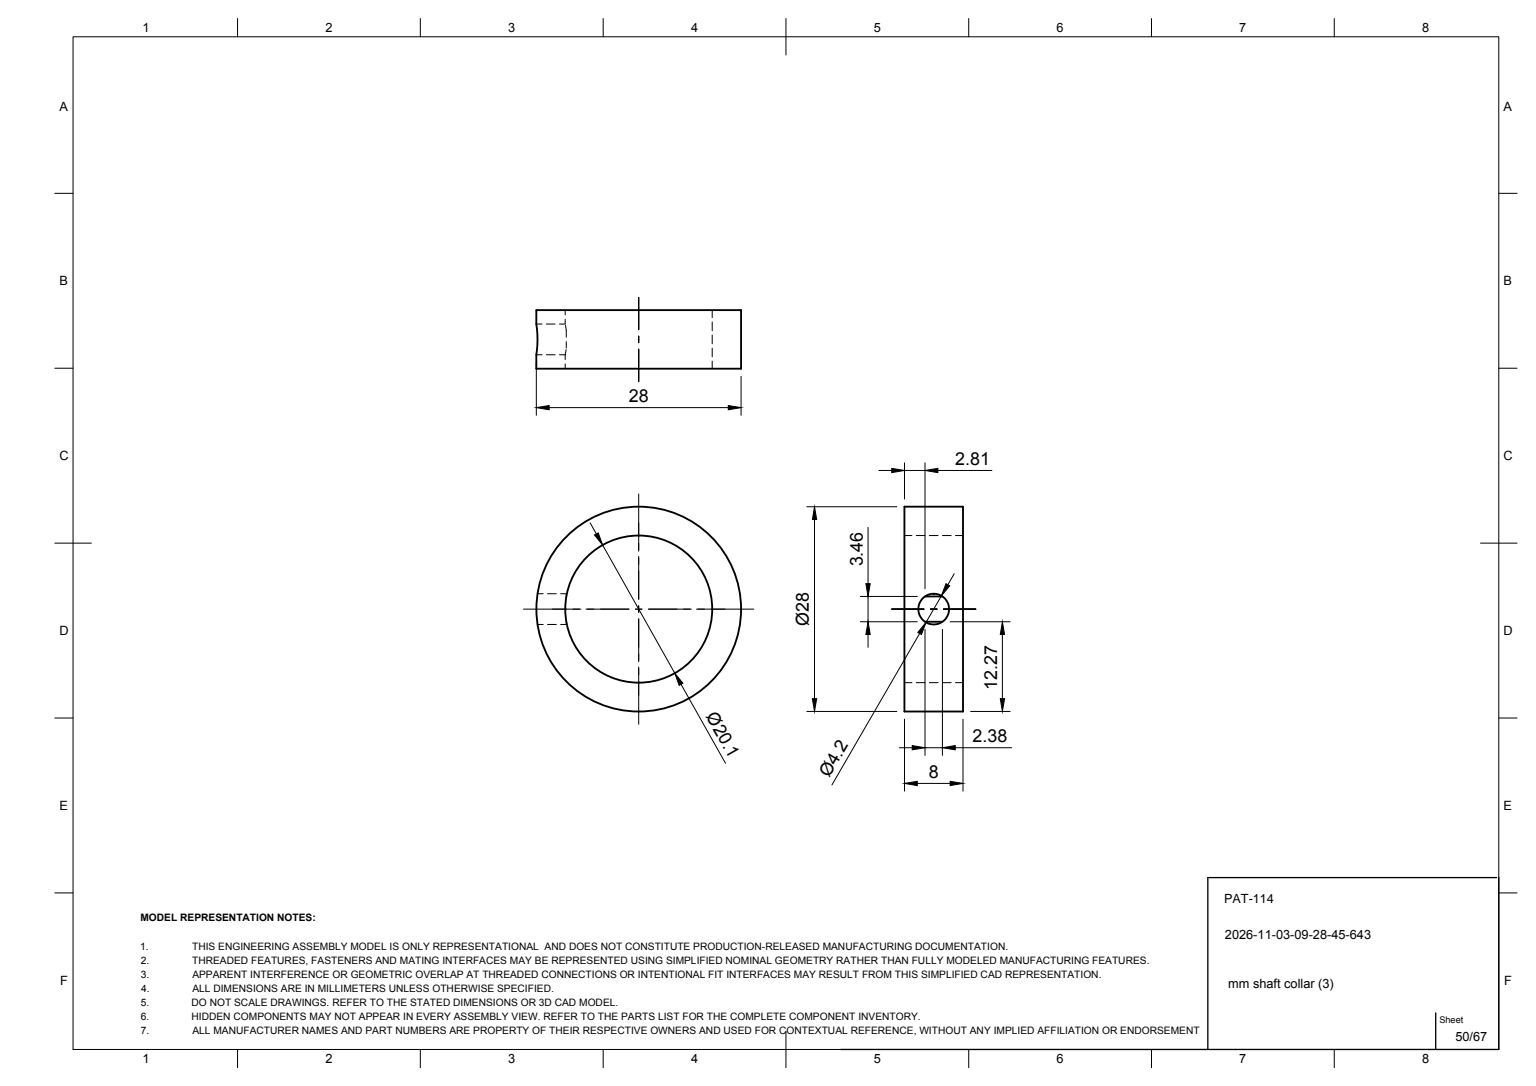
ISO-10303-21;
HEADER;
/* Generated by software containing ST-Developer
 * from STEP Tools, Inc. (www.steptools.com) 
 */

FILE_DESCRIPTION(
/* description */ ('Two-stage gear reducer in split housing'),
/* implementation_level */ '2;1');

FILE_NAME(
/* name */ 'mm shaft collar (3).step',
/* time_stamp */ '2026-10-28T03:22:31-07:00',
/* author */ (''),
/* organization */ (''),
/* preprocessor_version */ 'ST-DEVELOPER v20.2',
/* originating_system */ 'Autodesk Translation Framework v15.17.0.0',
/* authorisation */ '');

FILE_SCHEMA (('AUTOMOTIVE_DESIGN { 1 0 10303 214 3 1 1 }'));
ENDSEC;

DATA;
#10=MECHANICAL_DESIGN_GEOMETRIC_PRESENTATION_REPRESENTATION('',(#1288),#73366);
#975=B_SPLINE_CURVE_WITH_KNOTS('',3,(#37499,#37500,#37501,#37502,#37503,
#37504,#37505,#37506,#37507,#37508,#37509,#37510,#37511,#37512),
 .UNSPECIFIED.,.F.,.F.,(4,2,2,2,2,2,4),(0.75600573798703,0.793568827564647,
0.872922520054202,0.952276212543757,1.03162990503331,1.11098359752287,1.14854668710048),
 .UNSPECIFIED.);
#976=B_SPLINE_CURVE_WITH_KNOTS('',3,(#37518,#37519,#37520,#37521,#37522,
#37523,#37524,#37525,#37526,#37527,#37528,#37529,#37530,#37531,#37532,#37533,
#37534,#37535),.UNSPECIFIED.,.F.,.F.,(4,2,2,2,2,2,2,2,4),(0.,0.0792334805614374,
0.158466961122875,0.237699060165218,0.31693115920756,0.396163258249903,
0.475395357292246,0.554628837853684,0.633862318415121),.UNSPECIFIED.);
#977=B_SPLINE_CURVE_WITH_KNOTS('',3,(#37536,#37537,#37538,#37539,#37540,
#37541,#37542,#37543,#37544,#37545,#37546,#37547,#37548,#37549,#37550,#37551,
#37552,#37553),.UNSPECIFIED.,.F.,.F.,(4,2,2,2,2,2,2,2,4),(0.633862318415121,
0.713095798976559,0.792329279537996,0.871561378580339,0.950793477622681,
1.03002557666502,1.10925767570737,1.1884911562688,1.26772463683024),
 .UNSPECIFIED.);
#978=B_SPLINE_CURVE_WITH_KNOTS('',3,(#37556,#37557,#37558,#37559,#37560,
#37561,#37562,#37563,#37564,#37565,#37566,#37567,#37568,#37569),
 .UNSPECIFIED.,.F.,.F.,(4,2,2,2,2,2,4),(0.121154929624528,0.158718019202143,
0.238071711691698,0.317425404181252,0.396779096670807,0.476132789160361,
0.513695878737976),.UNSPECIFIED.);
#1161=SHAPE_REPRESENTATION_RELATIONSHIP('SRR','None',#73652,#1217);
#1217=ADVANCED_BREP_SHAPE_REPRESENTATION('',(#1357),#73348);
#1288=STYLED_ITEM('',(#73988),#1357);
#1357=MANIFOLD_SOLID_BREP('Body1',#16178);
#1564=FACE_BOUND('',#3679,.T.);
#1565=FACE_BOUND('',#3681,.T.);
#1566=FACE_BOUND('',#3683,.T.);
#1567=FACE_BOUND('',#3685,.T.);
#1874=PLANE('',#17985);
#1875=PLANE('',#17990);
#1876=PLANE('',#17997);
#1877=PLANE('',#17998);
#2572=FACE_OUTER_BOUND('',#3675,.T.);
#2573=FACE_OUTER_BOUND('',#3676,.T.);
#2574=FACE_OUTER_BOUND('',#3677,.T.);
#2575=FACE_OUTER_BOUND('',#3678,.T.);
#2576=FACE_OUTER_BOUND('',#3680,.T.);
#2577=FACE_OUTER_BOUND('',#3682,.T.);
#2578=FACE_OUTER_BOUND('',#3684,.T.);
#3675=EDGE_LOOP('',(#13075,#13076));
#3676=EDGE_LOOP('',(#13077,#13078,#13079,#13080,#13081,#13082,#13083,#13084,
#13085));
#3677=EDGE_LOOP('',(#13086,#13087,#13088));
#3678=EDGE_LOOP('',(#13089,#13090,#13091,#13092));
#3679=EDGE_LOOP('',(#13093,#13094,#13095,#13096));
#3680=EDGE_LOOP('',(#13097,#13098,#13099,#13100));
#3681=EDGE_LOOP('',(#13101,#13102));
#3682=EDGE_LOOP('',(#13103));
#3683=EDGE_LOOP('',(#13104));
#3684=EDGE_LOOP('',(#13105));
#3685=EDGE_LOOP('',(#13106));
#4689=LINE('',#37495,#5713);
#4690=LINE('',#37516,#5714);
#4691=LINE('',#37571,#5715);
#4692=LINE('',#37576,#5716);
#4693=LINE('',#37582,#5717);
#5713=VECTOR('',#21439,1.);
#5714=VECTOR('',#21446,0.21);
#5715=VECTOR('',#21451,1.);
#5716=VECTOR('',#21456,1.005);
#5717=VECTOR('',#21463,1.4);
#6631=CIRCLE('',#17986,0.21);
#6632=CIRCLE('',#17988,0.21);
#6633=CIRCLE('',#17989,0.21);
#6634=CIRCLE('',#17992,1.005);
#6635=CIRCLE('',#17993,1.005);
#6636=CIRCLE('',#17995,1.4);
#6637=CIRCLE('',#17996,1.4);
#7696=VERTEX_POINT('',#37493);
#7697=VERTEX_POINT('',#37494);
#7698=VERTEX_POINT('',#37498);
#7699=VERTEX_POINT('',#37513);
#7700=VERTEX_POINT('',#37515);
#7701=VERTEX_POINT('',#37517);
#7702=VERTEX_POINT('',#37554);
#7703=VERTEX_POINT('',#37573);
#7704=VERTEX_POINT('',#37575);
#7705=VERTEX_POINT('',#37579);
#7706=VERTEX_POINT('',#37581);
#9591=EDGE_CURVE('',#7696,#7697,#4689,.T.);
#9592=EDGE_CURVE('',#7696,#7697,#6631,.T.);
#9593=EDGE_CURVE('',#7698,#7696,#975,.T.);
#9594=EDGE_CURVE('',#7699,#7698,#6632,.T.);
#9595=EDGE_CURVE('',#7699,#7700,#4690,.T.);
#9596=EDGE_CURVE('',#7701,#7700,#976,.T.);
#9597=EDGE_CURVE('',#7700,#7701,#977,.T.);
#9598=EDGE_CURVE('',#7702,#7699,#6633,.T.);
#9599=EDGE_CURVE('',#7697,#7702,#978,.T.);
#9600=EDGE_CURVE('',#7702,#7698,#4691,.T.);
#9601=EDGE_CURVE('',#7703,#7703,#6634,.T.);
#9602=EDGE_CURVE('',#7703,#7704,#4692,.T.);
#9603=EDGE_CURVE('',#7704,#7704,#6635,.T.);
#9604=EDGE_CURVE('',#7705,#7705,#6636,.T.);
#9605=EDGE_CURVE('',#7705,#7706,#4693,.T.);
#9606=EDGE_CURVE('',#7706,#7706,#6637,.T.);
#13075=ORIENTED_EDGE('',*,*,#9591,.F.);
#13076=ORIENTED_EDGE('',*,*,#9592,.T.);
#13077=ORIENTED_EDGE('',*,*,#9593,.F.);
#13078=ORIENTED_EDGE('',*,*,#9594,.F.);
#13079=ORIENTED_EDGE('',*,*,#9595,.T.);
#13080=ORIENTED_EDGE('',*,*,#9596,.F.);
#13081=ORIENTED_EDGE('',*,*,#9597,.F.);
#13082=ORIENTED_EDGE('',*,*,#9595,.F.);
#13083=ORIENTED_EDGE('',*,*,#9598,.F.);
#13084=ORIENTED_EDGE('',*,*,#9599,.F.);
#13085=ORIENTED_EDGE('',*,*,#9592,.F.);
#13086=ORIENTED_EDGE('',*,*,#9600,.F.);
#13087=ORIENTED_EDGE('',*,*,#9598,.T.);
#13088=ORIENTED_EDGE('',*,*,#9594,.T.);
#13089=ORIENTED_EDGE('',*,*,#9601,.F.);
#13090=ORIENTED_EDGE('',*,*,#9602,.T.);
#13091=ORIENTED_EDGE('',*,*,#9603,.T.);
#13092=ORIENTED_EDGE('',*,*,#9602,.F.);
#13093=ORIENTED_EDGE('',*,*,#9599,.T.);
#13094=ORIENTED_EDGE('',*,*,#9600,.T.);
#13095=ORIENTED_EDGE('',*,*,#9593,.T.);
#13096=ORIENTED_EDGE('',*,*,#9591,.T.);
#13097=ORIENTED_EDGE('',*,*,#9604,.F.);
#13098=ORIENTED_EDGE('',*,*,#9605,.T.);
#13099=ORIENTED_EDGE('',*,*,#9606,.T.);
#13100=ORIENTED_EDGE('',*,*,#9605,.F.);
#13101=ORIENTED_EDGE('',*,*,#9596,.T.);
#13102=ORIENTED_EDGE('',*,*,#9597,.T.);
#13103=ORIENTED_EDGE('',*,*,#9604,.T.);
#13104=ORIENTED_EDGE('',*,*,#9601,.T.);
#13105=ORIENTED_EDGE('',*,*,#9606,.F.);
#13106=ORIENTED_EDGE('',*,*,#9603,.F.);
#15116=CYLINDRICAL_SURFACE('',#17987,0.21);
#15117=CYLINDRICAL_SURFACE('',#17991,1.005);
#15118=CYLINDRICAL_SURFACE('',#17994,1.4);
#15779=ADVANCED_FACE('',(#2572),#1874,.T.);
#15780=ADVANCED_FACE('',(#2573),#15116,.F.);
#15781=ADVANCED_FACE('',(#2574),#1875,.T.);
#15782=ADVANCED_FACE('',(#2575,#1564),#15117,.F.);
#15783=ADVANCED_FACE('',(#2576,#1565),#15118,.T.);
#15784=ADVANCED_FACE('',(#2577,#1566),#1876,.T.);
#15785=ADVANCED_FACE('',(#2578,#1567),#1877,.F.);
#16178=CLOSED_SHELL('',(#15779,#15780,#15781,#15782,#15783,#15784,#15785));
#17984=AXIS2_PLACEMENT_3D('',#37491,#21435,#21436);
#17985=AXIS2_PLACEMENT_3D('',#37492,#21437,#21438);
#17986=AXIS2_PLACEMENT_3D('',#37496,#21440,#21441);
#17987=AXIS2_PLACEMENT_3D('',#37497,#21442,#21443);
#17988=AXIS2_PLACEMENT_3D('',#37514,#21444,#21445);
#17989=AXIS2_PLACEMENT_3D('',#37555,#21447,#21448);
#17990=AXIS2_PLACEMENT_3D('',#37570,#21449,#21450);
#17991=AXIS2_PLACEMENT_3D('',#37572,#21452,#21453);
#17992=AXIS2_PLACEMENT_3D('',#37574,#21454,#21455);
#17993=AXIS2_PLACEMENT_3D('',#37577,#21457,#21458);
#17994=AXIS2_PLACEMENT_3D('',#37578,#21459,#21460);
#17995=AXIS2_PLACEMENT_3D('',#37580,#21461,#21462);
#17996=AXIS2_PLACEMENT_3D('',#37583,#21464,#21465);
#17997=AXIS2_PLACEMENT_3D('',#37584,#21466,#21467);
#17998=AXIS2_PLACEMENT_3D('',#37585,#21468,#21469);
#21435=DIRECTION('axis',(0.,0.,1.));
#21436=DIRECTION('refdir',(1.,0.,0.));
#21437=DIRECTION('center_axis',(0.,0.,1.));
#21438=DIRECTION('ref_axis',(1.,0.,0.));
#21439=DIRECTION('',(0.,1.,0.));
#21440=DIRECTION('center_axis',(0.,0.,1.));
#21441=DIRECTION('ref_axis',(1.,0.,0.));
#21442=DIRECTION('center_axis',(0.,0.,1.));
#21443=DIRECTION('ref_axis',(1.,0.,0.));
#21444=DIRECTION('center_axis',(0.,0.,1.));
#21445=DIRECTION('ref_axis',(1.,0.,0.));
#21446=DIRECTION('',(0.,0.,1.));
#21447=DIRECTION('center_axis',(0.,0.,1.));
#21448=DIRECTION('ref_axis',(1.,0.,0.));
#21449=DIRECTION('center_axis',(0.,0.,1.));
#21450=DIRECTION('ref_axis',(1.,0.,0.));
#21451=DIRECTION('',(0.,-1.,0.));
#21452=DIRECTION('center_axis',(0.,1.,0.));
#21453=DIRECTION('ref_axis',(1.,0.,0.));
#21454=DIRECTION('center_axis',(0.,-1.,0.));
#21455=DIRECTION('ref_axis',(1.,0.,0.));
#21456=DIRECTION('',(0.,-1.,0.));
#21457=DIRECTION('center_axis',(0.,-1.,0.));
#21458=DIRECTION('ref_axis',(1.,0.,0.));
#21459=DIRECTION('center_axis',(0.,1.,0.));
#21460=DIRECTION('ref_axis',(1.,0.,0.));
#21461=DIRECTION('center_axis',(0.,1.,0.));
#21462=DIRECTION('ref_axis',(1.,0.,0.));
#21463=DIRECTION('',(0.,-1.,0.));
#21464=DIRECTION('center_axis',(0.,1.,0.));
#21465=DIRECTION('ref_axis',(1.,0.,0.));
#21466=DIRECTION('center_axis',(0.,1.,0.));
#21467=DIRECTION('ref_axis',(1.,0.,0.));
#21468=DIRECTION('center_axis',(0.,1.,0.));
#21469=DIRECTION('ref_axis',(1.,0.,0.));
#37491=CARTESIAN_POINT('',(0.,0.,0.));
#37492=CARTESIAN_POINT('Origin',(6.,8.2,10.99));
#37493=CARTESIAN_POINT('',(6.17298843892005,8.08094119100208,10.99));
#37494=CARTESIAN_POINT('',(6.17298843892005,8.31905880899792,10.99));
#37495=CARTESIAN_POINT('',(6.17298843892005,7.8,10.99));
#37496=CARTESIAN_POINT('Origin',(6.,8.2,10.99));
#37497=CARTESIAN_POINT('Origin',(6.,8.2,10.99));
#37498=CARTESIAN_POINT('',(5.82701156107995,8.08094119100208,10.99));
#37499=CARTESIAN_POINT('Ctrl Pts',(5.82701156107995,8.08094119100207,10.99));
#37500=CARTESIAN_POINT('Ctrl Pts',(5.83440513468869,8.0701985776047,10.9912919219764));
#37501=CARTESIAN_POINT('Ctrl Pts',(5.8427028612744,8.06031229062725,10.992653949439));
#37502=CARTESIAN_POINT('Ctrl Pts',(5.87010792615492,8.03290722574673,10.9967480843909));
#37503=CARTESIAN_POINT('Ctrl Pts',(5.89366983224071,8.01675794366705,10.9996958932764));
#37504=CARTESIAN_POINT('Ctrl Pts',(5.94538709536759,7.99530220603509,11.0038502947236));
#37505=CARTESIAN_POINT('Ctrl Pts',(5.97354876917015,7.99,11.005));
#37506=CARTESIAN_POINT('Ctrl Pts',(6.02645123082985,7.99,11.005));
#37507=CARTESIAN_POINT('Ctrl Pts',(6.05461290463241,7.99530220603509,11.0038502947236));
#37508=CARTESIAN_POINT('Ctrl Pts',(6.10633016775928,8.01675794366705,10.9996958932764));
#37509=CARTESIAN_POINT('Ctrl Pts',(6.12989207384508,8.03290722574673,10.9967480843909));
#37510=CARTESIAN_POINT('Ctrl Pts',(6.1572971387256,8.06031229062725,10.992653949439));
#37511=CARTESIAN_POINT('Ctrl Pts',(6.16559486531131,8.0701985776047,10.9912919219764));
#37512=CARTESIAN_POINT('Ctrl Pts',(6.17298843892005,8.08094119100208,10.99));
#37513=CARTESIAN_POINT('',(5.79,8.2,10.99));
#37514=CARTESIAN_POINT('Origin',(6.,8.2,10.99));
#37515=CARTESIAN_POINT('',(5.79,8.2,11.38416039533));
#37516=CARTESIAN_POINT('',(5.79,8.2,10.99));
#37517=CARTESIAN_POINT('',(6.21,8.2,11.38416039533));
#37518=CARTESIAN_POINT('Ctrl Pts',(6.21,8.2,11.38416039533));
#37519=CARTESIAN_POINT('Ctrl Pts',(6.21,8.17358883981285,11.38416039533));
#37520=CARTESIAN_POINT('Ctrl Pts',(6.20471354911189,8.1454449403829,11.3849944296993));
#37521=CARTESIAN_POINT('Ctrl Pts',(6.18326999585849,8.09371735000826,11.3879947099895));
#37522=CARTESIAN_POINT('Ctrl Pts',(6.16711503760643,8.07013018950807,11.3901162943626));
#37523=CARTESIAN_POINT('Ctrl Pts',(6.12987013519678,8.03288528709843,11.394089123191));
#37524=CARTESIAN_POINT('Ctrl Pts',(6.10628283459019,8.01673007414492,11.3962002442067));
#37525=CARTESIAN_POINT('Ctrl Pts',(6.05455476560391,7.99528633552708,11.3991765222353));
#37526=CARTESIAN_POINT('Ctrl Pts',(6.02641069968078,7.99,11.4));
#37527=CARTESIAN_POINT('Ctrl Pts',(5.97358930031922,7.99,11.4));
#37528=CARTESIAN_POINT('Ctrl Pts',(5.94544523439609,7.99528633552708,11.3991765222353));
#37529=CARTESIAN_POINT('Ctrl Pts',(5.89371716540981,8.01673007414492,11.3962002442067));
#37530=CARTESIAN_POINT('Ctrl Pts',(5.87012986480322,8.03288528709843,11.394089123191));
#37531=CARTESIAN_POINT('Ctrl Pts',(5.83288496239357,8.07013018950807,11.3901162943626));
#37532=CARTESIAN_POINT('Ctrl Pts',(5.81673000414151,8.09371735000826,11.3879947099895));
#37533=CARTESIAN_POINT('Ctrl Pts',(5.79528645088811,8.1454449403829,11.3849944296993));
#37534=CARTESIAN_POINT('Ctrl Pts',(5.79,8.17358883981285,11.38416039533));
#37535=CARTESIAN_POINT('Ctrl Pts',(5.79,8.2,11.38416039533));
#37536=CARTESIAN_POINT('Ctrl Pts',(5.79,8.2,11.38416039533));
#37537=CARTESIAN_POINT('Ctrl Pts',(5.79,8.22641116018715,11.38416039533));
#37538=CARTESIAN_POINT('Ctrl Pts',(5.79528645088811,8.2545550596171,11.3849944296993));
#37539=CARTESIAN_POINT('Ctrl Pts',(5.81673000414151,8.30628264999174,11.3879947099895));
#37540=CARTESIAN_POINT('Ctrl Pts',(5.83288496239357,8.32986981049192,11.3901162943626));
#37541=CARTESIAN_POINT('Ctrl Pts',(5.87012986480322,8.36711471290156,11.394089123191));
#37542=CARTESIAN_POINT('Ctrl Pts',(5.89371716540981,8.38326992585508,11.3962002442067));
#37543=CARTESIAN_POINT('Ctrl Pts',(5.94544523439609,8.40471366447292,11.3991765222353));
#37544=CARTESIAN_POINT('Ctrl Pts',(5.97358930031922,8.41,11.4));
#37545=CARTESIAN_POINT('Ctrl Pts',(6.02641069968078,8.41,11.4));
#37546=CARTESIAN_POINT('Ctrl Pts',(6.05455476560391,8.40471366447292,11.3991765222353));
#37547=CARTESIAN_POINT('Ctrl Pts',(6.10628283459019,8.38326992585508,11.3962002442067));
#37548=CARTESIAN_POINT('Ctrl Pts',(6.12987013519678,8.36711471290156,11.394089123191));
#37549=CARTESIAN_POINT('Ctrl Pts',(6.16711503760642,8.32986981049192,11.3901162943626));
#37550=CARTESIAN_POINT('Ctrl Pts',(6.18326999585849,8.30628264999174,11.3879947099895));
#37551=CARTESIAN_POINT('Ctrl Pts',(6.2047135491119,8.2545550596171,11.3849944296993));
#37552=CARTESIAN_POINT('Ctrl Pts',(6.21,8.22641116018714,11.38416039533));
#37553=CARTESIAN_POINT('Ctrl Pts',(6.21,8.2,11.38416039533));
#37554=CARTESIAN_POINT('',(5.82701156107995,8.31905880899792,10.99));
#37555=CARTESIAN_POINT('Origin',(6.,8.2,10.99));
#37556=CARTESIAN_POINT('Ctrl Pts',(6.17298843892005,8.31905880899792,10.99));
#37557=CARTESIAN_POINT('Ctrl Pts',(6.16559486531131,8.3298014223953,10.9912919219764));
#37558=CARTESIAN_POINT('Ctrl Pts',(6.1572971387256,8.33968770937275,10.992653949439));
#37559=CARTESIAN_POINT('Ctrl Pts',(6.12989207384508,8.36709277425327,10.9967480843909));
#37560=CARTESIAN_POINT('Ctrl Pts',(6.10633016775928,8.38324205633295,10.9996958932764));
#37561=CARTESIAN_POINT('Ctrl Pts',(6.05461290463241,8.40469779396491,11.0038502947236));
#37562=CARTESIAN_POINT('Ctrl Pts',(6.02645123082985,8.41,11.005));
#37563=CARTESIAN_POINT('Ctrl Pts',(5.97354876917015,8.41,11.005));
#37564=CARTESIAN_POINT('Ctrl Pts',(5.94538709536759,8.40469779396491,11.0038502947236));
#37565=CARTESIAN_POINT('Ctrl Pts',(5.89366983224072,8.38324205633295,10.9996958932764));
#37566=CARTESIAN_POINT('Ctrl Pts',(5.87010792615492,8.36709277425327,10.9967480843909));
#37567=CARTESIAN_POINT('Ctrl Pts',(5.8427028612744,8.33968770937275,10.992653949439));
#37568=CARTESIAN_POINT('Ctrl Pts',(5.83440513468869,8.3298014223953,10.9912919219764));
#37569=CARTESIAN_POINT('Ctrl Pts',(5.82701156107995,8.31905880899792,10.99));
#37570=CARTESIAN_POINT('Origin',(6.,8.2,10.99));
#37571=CARTESIAN_POINT('',(5.82701156107995,7.8,10.99));
#37572=CARTESIAN_POINT('Origin',(6.,7.8,10.));
#37573=CARTESIAN_POINT('',(4.995,8.6,10.));
#37574=CARTESIAN_POINT('Origin',(6.,8.6,10.));
#37575=CARTESIAN_POINT('',(4.995,7.8,10.));
#37576=CARTESIAN_POINT('',(4.995,7.8,10.));
#37577=CARTESIAN_POINT('Origin',(6.,7.8,10.));
#37578=CARTESIAN_POINT('Origin',(6.,7.8,10.));
#37579=CARTESIAN_POINT('',(4.6,8.6,10.));
#37580=CARTESIAN_POINT('Origin',(6.,8.6,10.));
#37581=CARTESIAN_POINT('',(4.6,7.8,10.));
#37582=CARTESIAN_POINT('',(4.6,7.8,10.));
#37583=CARTESIAN_POINT('Origin',(6.,7.8,10.));
#37584=CARTESIAN_POINT('Origin',(6.,8.6,10.));
#37585=CARTESIAN_POINT('Origin',(6.,7.8,10.));
#73284=UNCERTAINTY_MEASURE_WITH_UNIT(LENGTH_MEASURE(0.001),#73367,
'DISTANCE_ACCURACY_VALUE',
'Maximum model space distance between geometric entities at asserted c
onnectivities');
#73302=UNCERTAINTY_MEASURE_WITH_UNIT(LENGTH_MEASURE(0.001),#73367,
'DISTANCE_ACCURACY_VALUE',
'Maximum model space distance between geometric entities at asserted c
onnectivities');
#73348=(
GEOMETRIC_REPRESENTATION_CONTEXT(3)
GLOBAL_UNCERTAINTY_ASSIGNED_CONTEXT((#73284))
GLOBAL_UNIT_ASSIGNED_CONTEXT((#73367,#73369,#73370))
REPRESENTATION_CONTEXT('','3D')
);
#73366=(
GEOMETRIC_REPRESENTATION_CONTEXT(3)
GLOBAL_UNCERTAINTY_ASSIGNED_CONTEXT((#73302))
GLOBAL_UNIT_ASSIGNED_CONTEXT((#73367,#73369,#73370))
REPRESENTATION_CONTEXT('','3D')
);
#73367=(
LENGTH_UNIT()
NAMED_UNIT(*)
SI_UNIT(.CENTI.,.METRE.)
);
#73369=(
NAMED_UNIT(*)
PLANE_ANGLE_UNIT()
SI_UNIT($,.RADIAN.)
);
#73370=(
NAMED_UNIT(*)
SI_UNIT($,.STERADIAN.)
SOLID_ANGLE_UNIT()
);
#73416=SHAPE_DEFINITION_REPRESENTATION(#73549,#73652);
#73549=PRODUCT_DEFINITION_SHAPE('',$,#73716);
#73652=SHAPE_REPRESENTATION('',(#17984),#73348);
#73670=PRODUCT_DEFINITION_CONTEXT('part definition',#73861,'design');
#73716=PRODUCT_DEFINITION('mm shaft collar (3)','mm shaft collar (3)',#73779,
#73670);
#73779=PRODUCT_DEFINITION_FORMATION('',$,#73908);
#73861=APPLICATION_CONTEXT(
'Core Data for Automotive Mechanical Design Process');
#73862=PRODUCT_CONTEXT('part definition',#73861,'mechanical');
#73908=PRODUCT('mm shaft collar (3)','mm shaft collar (3)',
'mm shaft collar (3)',(#73862));
#73982=COLOUR_RGB('Grey',0.48,0.52,0.57);
#73983=FILL_AREA_STYLE_COLOUR('',#73982);
#73984=FILL_AREA_STYLE('',(#73983));
#73985=SURFACE_STYLE_FILL_AREA(#73984);
#73986=SURFACE_SIDE_STYLE('',(#73985));
#73987=SURFACE_STYLE_USAGE(.BOTH.,#73986);
#73988=PRESENTATION_STYLE_ASSIGNMENT((#73987));
ENDSEC;
END-ISO-10303-21;
